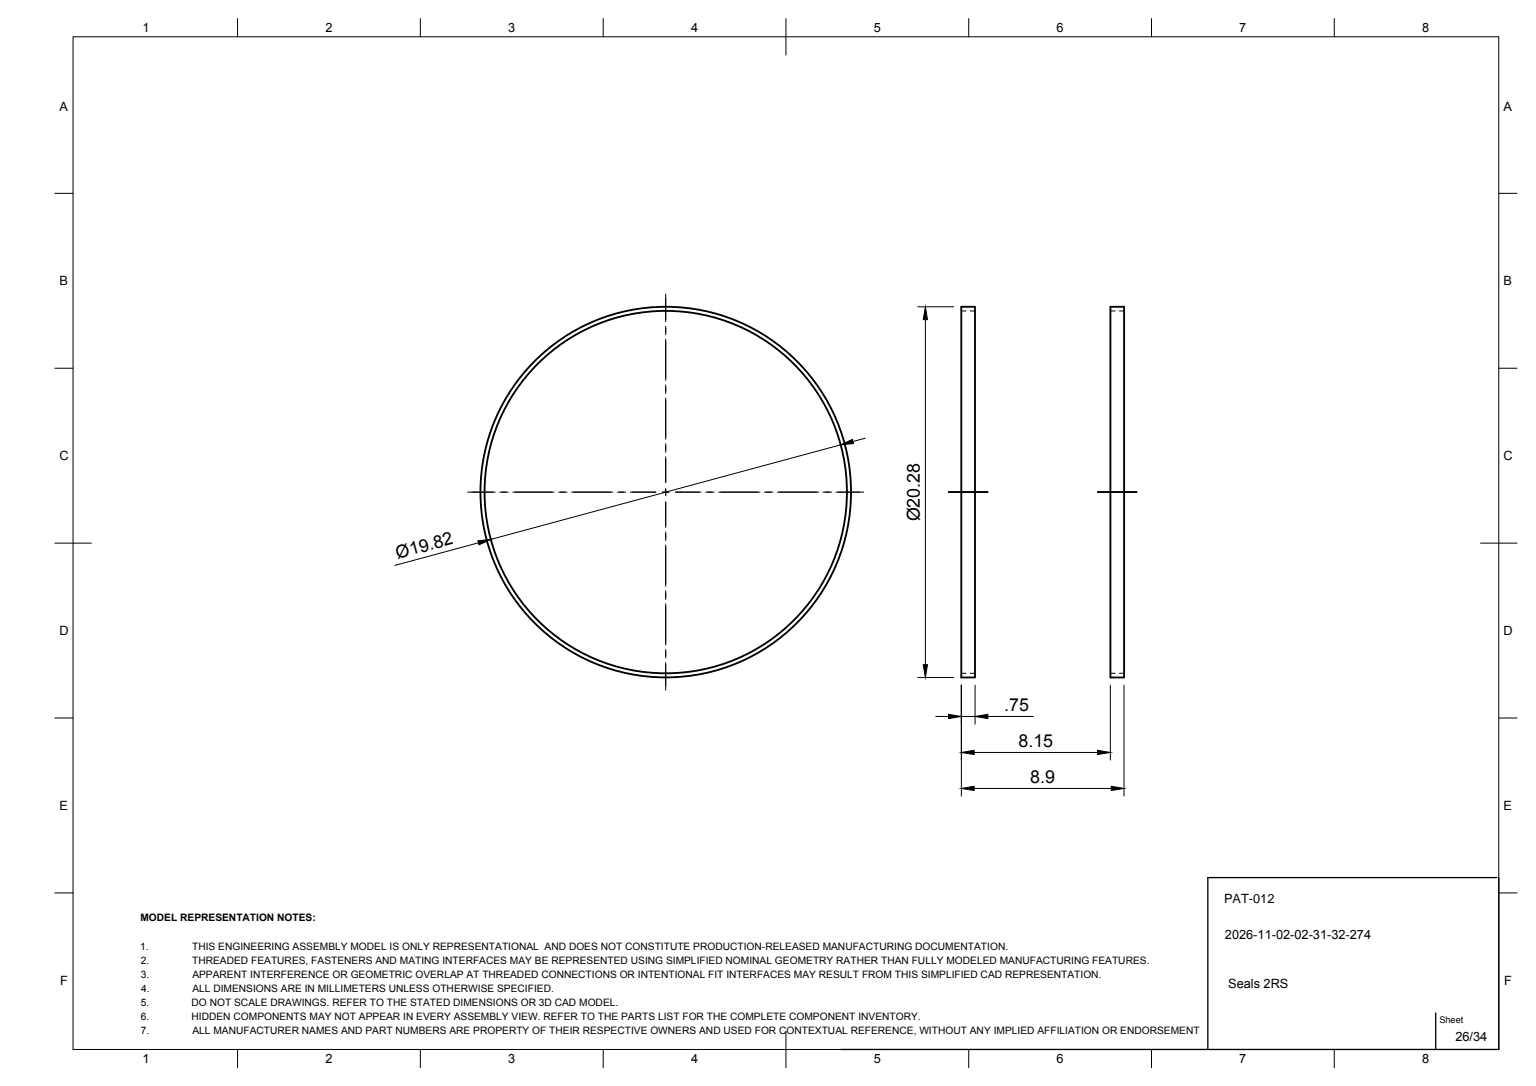
ISO-10303-21;
HEADER;
/* Generated by software containing ST-Developer
 * from STEP Tools, Inc. (www.steptools.com) 
 */

FILE_DESCRIPTION(
/* description */ ('Belt tensioner idler arm'),
/* implementation_level */ '2;1');

FILE_NAME(
/* name */ 'Seals 2RS.step',
/* time_stamp */ '2026-10-28T03:22:15-07:00',
/* author */ (''),
/* organization */ (''),
/* preprocessor_version */ 'ST-DEVELOPER v20.2',
/* originating_system */ 'Autodesk Translation Framework v15.17.0.0',
/* authorisation */ '');

FILE_SCHEMA (('AUTOMOTIVE_DESIGN { 1 0 10303 214 3 1 1 }'));
ENDSEC;

DATA;
#10=MECHANICAL_DESIGN_GEOMETRIC_PRESENTATION_REPRESENTATION('',(#476,#477),#12779);
#401=SHAPE_REPRESENTATION_RELATIONSHIP('SRR','None',#12949,#435);
#435=ADVANCED_BREP_SHAPE_REPRESENTATION('',(#516,#517),#12766);
#476=STYLED_ITEM('',(#13184),#516);
#477=STYLED_ITEM('',(#13184),#517);
#516=MANIFOLD_SOLID_BREP('Body1',#6212);
#517=MANIFOLD_SOLID_BREP('Body2',#6213);
#632=FACE_BOUND('',#1539,.T.);
#633=FACE_BOUND('',#1542,.T.);
#634=FACE_BOUND('',#1545,.T.);
#635=FACE_BOUND('',#1548,.T.);
#778=PLANE('',#7079);
#779=PLANE('',#7084);
#780=PLANE('',#7087);
#781=PLANE('',#7092);
#1066=FACE_OUTER_BOUND('',#1538,.T.);
#1067=FACE_OUTER_BOUND('',#1540,.T.);
#1068=FACE_OUTER_BOUND('',#1541,.T.);
#1069=FACE_OUTER_BOUND('',#1543,.T.);
#1070=FACE_OUTER_BOUND('',#1544,.T.);
#1071=FACE_OUTER_BOUND('',#1546,.T.);
#1072=FACE_OUTER_BOUND('',#1547,.T.);
#1073=FACE_OUTER_BOUND('',#1549,.T.);
#1538=EDGE_LOOP('',(#5048));
#1539=EDGE_LOOP('',(#5049));
#1540=EDGE_LOOP('',(#5050,#5051,#5052,#5053));
#1541=EDGE_LOOP('',(#5054));
#1542=EDGE_LOOP('',(#5055));
#1543=EDGE_LOOP('',(#5056,#5057,#5058,#5059));
#1544=EDGE_LOOP('',(#5060));
#1545=EDGE_LOOP('',(#5061));
#1546=EDGE_LOOP('',(#5062,#5063,#5064,#5065));
#1547=EDGE_LOOP('',(#5066));
#1548=EDGE_LOOP('',(#5067));
#1549=EDGE_LOOP('',(#5068,#5069,#5070,#5071));
#1919=LINE('',#11645,#2268);
#1920=LINE('',#11650,#2269);
#1921=LINE('',#11659,#2270);
#1922=LINE('',#11664,#2271);
#2268=VECTOR('',#8609,1.013815);
#2269=VECTOR('',#8616,0.991185);
#2270=VECTOR('',#8627,1.013815);
#2271=VECTOR('',#8634,0.991185);
#2626=CIRCLE('',#7080,1.013815);
#2627=CIRCLE('',#7081,0.991185);
#2628=CIRCLE('',#7083,1.013815);
#2629=CIRCLE('',#7085,0.991185);
#2630=CIRCLE('',#7088,1.013815);
#2631=CIRCLE('',#7089,0.991185);
#2632=CIRCLE('',#7091,1.013815);
#2633=CIRCLE('',#7093,0.991185);
#3092=VERTEX_POINT('',#11638);
#3093=VERTEX_POINT('',#11640);
#3094=VERTEX_POINT('',#11643);
#3095=VERTEX_POINT('',#11647);
#3096=VERTEX_POINT('',#11652);
#3097=VERTEX_POINT('',#11654);
#3098=VERTEX_POINT('',#11657);
#3099=VERTEX_POINT('',#11661);
#3779=EDGE_CURVE('',#3092,#3092,#2626,.T.);
#3780=EDGE_CURVE('',#3093,#3093,#2627,.T.);
#3781=EDGE_CURVE('',#3094,#3094,#2628,.T.);
#3782=EDGE_CURVE('',#3094,#3092,#1919,.T.);
#3783=EDGE_CURVE('',#3095,#3095,#2629,.T.);
#3784=EDGE_CURVE('',#3095,#3093,#1920,.T.);
#3785=EDGE_CURVE('',#3096,#3096,#2630,.T.);
#3786=EDGE_CURVE('',#3097,#3097,#2631,.T.);
#3787=EDGE_CURVE('',#3098,#3098,#2632,.T.);
#3788=EDGE_CURVE('',#3098,#3096,#1921,.T.);
#3789=EDGE_CURVE('',#3099,#3099,#2633,.T.);
#3790=EDGE_CURVE('',#3099,#3097,#1922,.T.);
#5048=ORIENTED_EDGE('',*,*,#3779,.F.);
#5049=ORIENTED_EDGE('',*,*,#3780,.T.);
#5050=ORIENTED_EDGE('',*,*,#3781,.F.);
#5051=ORIENTED_EDGE('',*,*,#3782,.T.);
#5052=ORIENTED_EDGE('',*,*,#3779,.T.);
#5053=ORIENTED_EDGE('',*,*,#3782,.F.);
#5054=ORIENTED_EDGE('',*,*,#3781,.T.);
#5055=ORIENTED_EDGE('',*,*,#3783,.F.);
#5056=ORIENTED_EDGE('',*,*,#3783,.T.);
#5057=ORIENTED_EDGE('',*,*,#3784,.T.);
#5058=ORIENTED_EDGE('',*,*,#3780,.F.);
#5059=ORIENTED_EDGE('',*,*,#3784,.F.);
#5060=ORIENTED_EDGE('',*,*,#3785,.F.);
#5061=ORIENTED_EDGE('',*,*,#3786,.T.);
#5062=ORIENTED_EDGE('',*,*,#3787,.F.);
#5063=ORIENTED_EDGE('',*,*,#3788,.T.);
#5064=ORIENTED_EDGE('',*,*,#3785,.T.);
#5065=ORIENTED_EDGE('',*,*,#3788,.F.);
#5066=ORIENTED_EDGE('',*,*,#3787,.T.);
#5067=ORIENTED_EDGE('',*,*,#3789,.F.);
#5068=ORIENTED_EDGE('',*,*,#3789,.T.);
#5069=ORIENTED_EDGE('',*,*,#3790,.T.);
#5070=ORIENTED_EDGE('',*,*,#3786,.F.);
#5071=ORIENTED_EDGE('',*,*,#3790,.F.);
#5742=CYLINDRICAL_SURFACE('',#7082,1.013815);
#5743=CYLINDRICAL_SURFACE('',#7086,0.991185);
#5744=CYLINDRICAL_SURFACE('',#7090,1.013815);
#5745=CYLINDRICAL_SURFACE('',#7094,0.991185);
#6043=ADVANCED_FACE('',(#1066,#632),#778,.T.);
#6044=ADVANCED_FACE('',(#1067),#5742,.T.);
#6045=ADVANCED_FACE('',(#1068,#633),#779,.T.);
#6046=ADVANCED_FACE('',(#1069),#5743,.F.);
#6047=ADVANCED_FACE('',(#1070,#634),#780,.T.);
#6048=ADVANCED_FACE('',(#1071),#5744,.T.);
#6049=ADVANCED_FACE('',(#1072,#635),#781,.T.);
#6050=ADVANCED_FACE('',(#1073),#5745,.F.);
#6212=CLOSED_SHELL('',(#6043,#6044,#6045,#6046));
#6213=CLOSED_SHELL('',(#6047,#6048,#6049,#6050));
#7078=AXIS2_PLACEMENT_3D('',#11636,#8597,#8598);
#7079=AXIS2_PLACEMENT_3D('',#11637,#8599,#8600);
#7080=AXIS2_PLACEMENT_3D('',#11639,#8601,#8602);
#7081=AXIS2_PLACEMENT_3D('',#11641,#8603,#8604);
#7082=AXIS2_PLACEMENT_3D('',#11642,#8605,#8606);
#7083=AXIS2_PLACEMENT_3D('',#11644,#8607,#8608);
#7084=AXIS2_PLACEMENT_3D('',#11646,#8610,#8611);
#7085=AXIS2_PLACEMENT_3D('',#11648,#8612,#8613);
#7086=AXIS2_PLACEMENT_3D('',#11649,#8614,#8615);
#7087=AXIS2_PLACEMENT_3D('',#11651,#8617,#8618);
#7088=AXIS2_PLACEMENT_3D('',#11653,#8619,#8620);
#7089=AXIS2_PLACEMENT_3D('',#11655,#8621,#8622);
#7090=AXIS2_PLACEMENT_3D('',#11656,#8623,#8624);
#7091=AXIS2_PLACEMENT_3D('',#11658,#8625,#8626);
#7092=AXIS2_PLACEMENT_3D('',#11660,#8628,#8629);
#7093=AXIS2_PLACEMENT_3D('',#11662,#8630,#8631);
#7094=AXIS2_PLACEMENT_3D('',#11663,#8632,#8633);
#8597=DIRECTION('axis',(0.,0.,1.));
#8598=DIRECTION('refdir',(1.,0.,0.));
#8599=DIRECTION('center_axis',(0.,1.,0.));
#8600=DIRECTION('ref_axis',(0.,0.,1.));
#8601=DIRECTION('center_axis',(0.,-1.,0.));
#8602=DIRECTION('ref_axis',(1.,0.,0.));
#8603=DIRECTION('center_axis',(0.,-1.,0.));
#8604=DIRECTION('ref_axis',(1.,0.,0.));
#8605=DIRECTION('center_axis',(0.,-1.,0.));
#8606=DIRECTION('ref_axis',(1.,0.,0.));
#8607=DIRECTION('center_axis',(0.,-1.,0.));
#8608=DIRECTION('ref_axis',(1.,0.,0.));
#8609=DIRECTION('',(0.,1.,0.));
#8610=DIRECTION('center_axis',(0.,-1.,0.));
#8611=DIRECTION('ref_axis',(0.,0.,-1.));
#8612=DIRECTION('center_axis',(0.,-1.,0.));
#8613=DIRECTION('ref_axis',(1.,0.,0.));
#8614=DIRECTION('center_axis',(0.,-1.,0.));
#8615=DIRECTION('ref_axis',(1.,0.,0.));
#8616=DIRECTION('',(0.,1.,0.));
#8617=DIRECTION('center_axis',(0.,1.,0.));
#8618=DIRECTION('ref_axis',(0.,0.,1.));
#8619=DIRECTION('center_axis',(0.,-1.,0.));
#8620=DIRECTION('ref_axis',(1.,0.,0.));
#8621=DIRECTION('center_axis',(0.,-1.,0.));
#8622=DIRECTION('ref_axis',(1.,0.,0.));
#8623=DIRECTION('center_axis',(0.,-1.,0.));
#8624=DIRECTION('ref_axis',(1.,0.,0.));
#8625=DIRECTION('center_axis',(0.,-1.,0.));
#8626=DIRECTION('ref_axis',(1.,0.,0.));
#8627=DIRECTION('',(0.,1.,0.));
#8628=DIRECTION('center_axis',(0.,-1.,0.));
#8629=DIRECTION('ref_axis',(0.,0.,-1.));
#8630=DIRECTION('center_axis',(0.,-1.,0.));
#8631=DIRECTION('ref_axis',(1.,0.,0.));
#8632=DIRECTION('center_axis',(0.,-1.,0.));
#8633=DIRECTION('ref_axis',(1.,0.,0.));
#8634=DIRECTION('',(0.,1.,0.));
#11636=CARTESIAN_POINT('',(0.,0.,0.));
#11637=CARTESIAN_POINT('Origin',(1.013815,0.445,0.));
#11638=CARTESIAN_POINT('',(-1.013815,0.445,-1.24156529467757E-16));
#11639=CARTESIAN_POINT('Origin',(0.,0.445,0.));
#11640=CARTESIAN_POINT('',(-0.991185,0.445,-1.21385153761287E-16));
#11641=CARTESIAN_POINT('Origin',(0.,0.445,0.));
#11642=CARTESIAN_POINT('Origin',(0.,0.4075,0.));
#11643=CARTESIAN_POINT('',(-1.013815,0.37,-1.24156529467757E-16));
#11644=CARTESIAN_POINT('Origin',(0.,0.37,0.));
#11645=CARTESIAN_POINT('',(-1.013815,0.4075,-1.24156529467757E-16));
#11646=CARTESIAN_POINT('Origin',(0.991185,0.37,0.));
#11647=CARTESIAN_POINT('',(-0.991185,0.37,-1.21385153761287E-16));
#11648=CARTESIAN_POINT('Origin',(0.,0.37,0.));
#11649=CARTESIAN_POINT('Origin',(0.,0.4075,0.));
#11650=CARTESIAN_POINT('',(-0.991185,0.4075,-1.21385153761287E-16));
#11651=CARTESIAN_POINT('Origin',(1.013815,-0.37,0.));
#11652=CARTESIAN_POINT('',(-1.013815,-0.37,-1.24156529467757E-16));
#11653=CARTESIAN_POINT('Origin',(0.,-0.37,0.));
#11654=CARTESIAN_POINT('',(-0.991185,-0.37,-1.21385153761287E-16));
#11655=CARTESIAN_POINT('Origin',(0.,-0.37,0.));
#11656=CARTESIAN_POINT('Origin',(0.,-0.4075,0.));
#11657=CARTESIAN_POINT('',(-1.013815,-0.445,-1.24156529467757E-16));
#11658=CARTESIAN_POINT('Origin',(0.,-0.445,0.));
#11659=CARTESIAN_POINT('',(-1.013815,-0.4075,-1.24156529467757E-16));
#11660=CARTESIAN_POINT('Origin',(0.991185,-0.445,0.));
#11661=CARTESIAN_POINT('',(-0.991185,-0.445,-1.21385153761287E-16));
#11662=CARTESIAN_POINT('Origin',(0.,-0.445,0.));
#11663=CARTESIAN_POINT('Origin',(0.,-0.4075,0.));
#11664=CARTESIAN_POINT('',(-0.991185,-0.4075,-1.21385153761287E-16));
#12726=UNCERTAINTY_MEASURE_WITH_UNIT(LENGTH_MEASURE(0.001),#12780,
'DISTANCE_ACCURACY_VALUE',
'Maximum model space distance between geometric entities at asserted c
onnectivities');
#12739=UNCERTAINTY_MEASURE_WITH_UNIT(LENGTH_MEASURE(0.001),#12780,
'DISTANCE_ACCURACY_VALUE',
'Maximum model space distance between geometric entities at asserted c
onnectivities');
#12766=(
GEOMETRIC_REPRESENTATION_CONTEXT(3)
GLOBAL_UNCERTAINTY_ASSIGNED_CONTEXT((#12726))
GLOBAL_UNIT_ASSIGNED_CONTEXT((#12780,#12782,#12783))
REPRESENTATION_CONTEXT('','3D')
);
#12779=(
GEOMETRIC_REPRESENTATION_CONTEXT(3)
GLOBAL_UNCERTAINTY_ASSIGNED_CONTEXT((#12739))
GLOBAL_UNIT_ASSIGNED_CONTEXT((#12780,#12782,#12783))
REPRESENTATION_CONTEXT('','3D')
);
#12780=(
LENGTH_UNIT()
NAMED_UNIT(*)
SI_UNIT(.CENTI.,.METRE.)
);
#12782=(
NAMED_UNIT(*)
PLANE_ANGLE_UNIT()
SI_UNIT($,.RADIAN.)
);
#12783=(
NAMED_UNIT(*)
SI_UNIT($,.STERADIAN.)
SOLID_ANGLE_UNIT()
);
#12810=SHAPE_DEFINITION_REPRESENTATION(#12849,#12949);
#12849=PRODUCT_DEFINITION_SHAPE('',$,#12989);
#12949=SHAPE_REPRESENTATION('',(#7078),#12766);
#12962=PRODUCT_DEFINITION_CONTEXT('part definition',#13081,'design');
#12989=PRODUCT_DEFINITION('Seals 2RS','Seals 2RS',#13028,#12962);
#13028=PRODUCT_DEFINITION_FORMATION('',$,#13109);
#13081=APPLICATION_CONTEXT(
'Core Data for Automotive Mechanical Design Process');
#13082=PRODUCT_CONTEXT('part definition',#13081,'mechanical');
#13109=PRODUCT('Seals 2RS','Seals 2RS','Seals 2RS',(#13082));
#13178=COLOUR_RGB('Grey',0.48,0.52,0.57);
#13179=FILL_AREA_STYLE_COLOUR('',#13178);
#13180=FILL_AREA_STYLE('',(#13179));
#13181=SURFACE_STYLE_FILL_AREA(#13180);
#13182=SURFACE_SIDE_STYLE('',(#13181));
#13183=SURFACE_STYLE_USAGE(.BOTH.,#13182);
#13184=PRESENTATION_STYLE_ASSIGNMENT((#13183));
ENDSEC;
END-ISO-10303-21;
